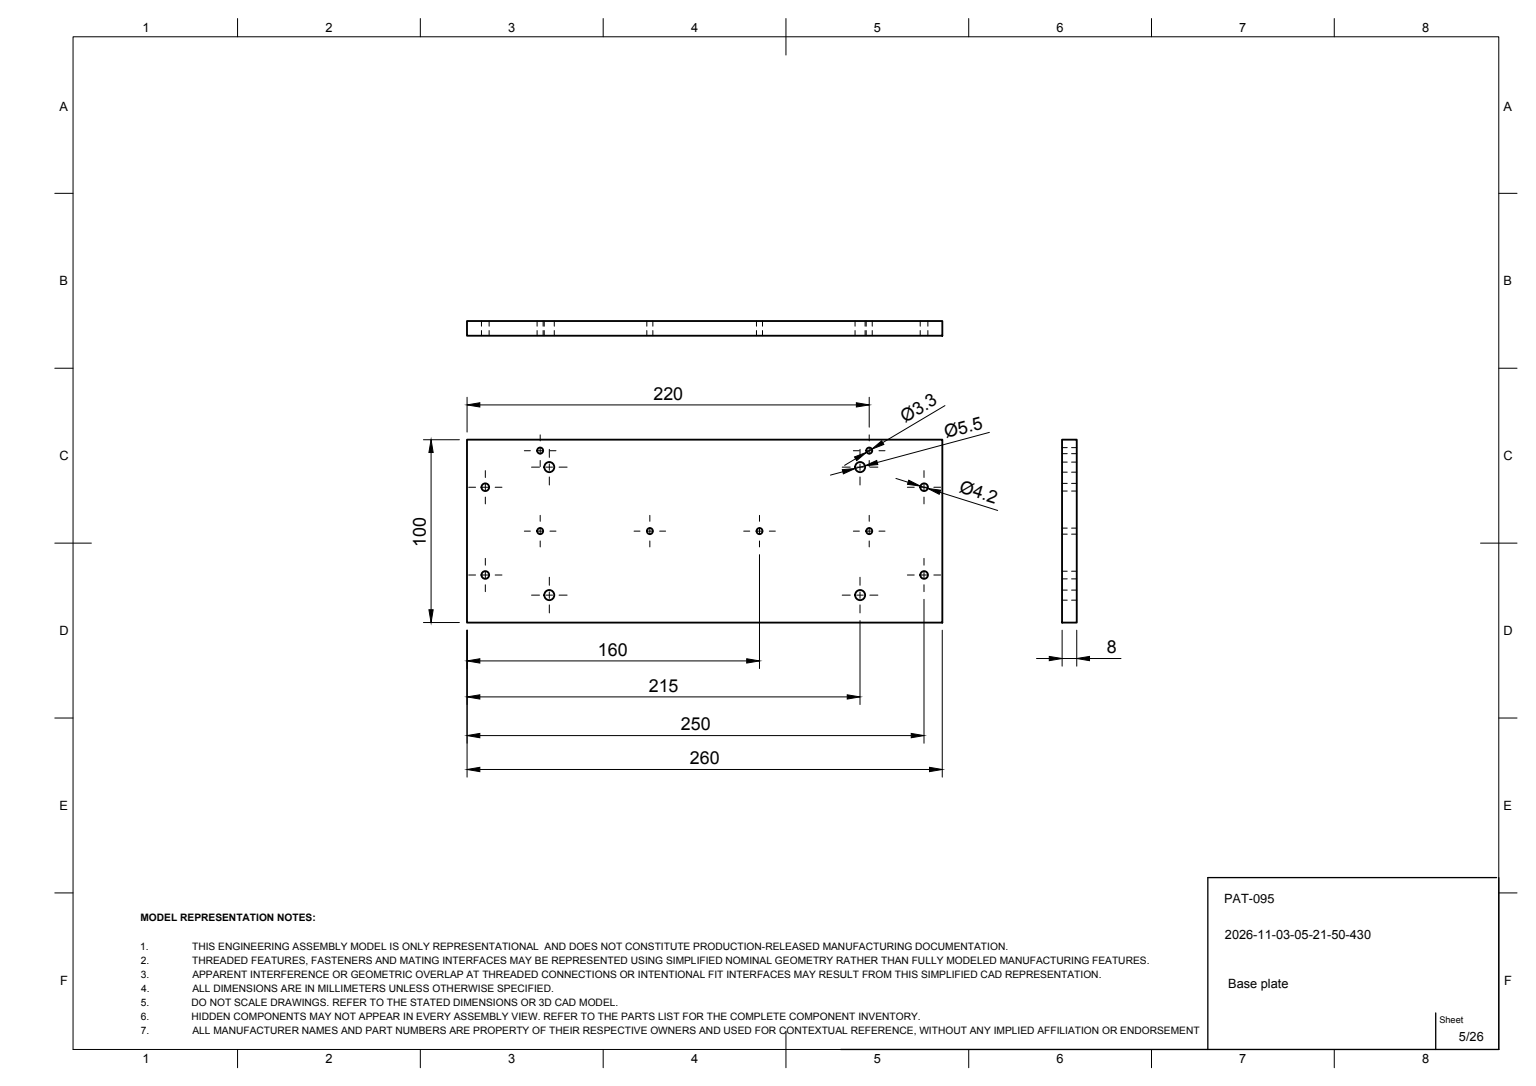
ISO-10303-21;
HEADER;
/* Generated by software containing ST-Developer
 * from STEP Tools, Inc. (www.steptools.com) 
 */

FILE_DESCRIPTION(
/* description */ ('Single-Axis Profile-Rail Linear Slide'),
/* implementation_level */ '2;1');

FILE_NAME(
/* name */ 'Base plate.step',
/* time_stamp */ '2026-10-27T10:47:43-07:00',
/* author */ (''),
/* organization */ (''),
/* preprocessor_version */ 'ST-DEVELOPER v20.2',
/* originating_system */ 'Autodesk Translation Framework v15.17.0.0',
/* authorisation */ '');

FILE_SCHEMA (('AUTOMOTIVE_DESIGN { 1 0 10303 214 3 1 1 }'));
ENDSEC;

DATA;
#10=MECHANICAL_DESIGN_GEOMETRIC_PRESENTATION_REPRESENTATION('',(#329),#14478);
#275=SHAPE_REPRESENTATION_RELATIONSHIP('SRR','None',#14605,#302);
#302=ADVANCED_BREP_SHAPE_REPRESENTATION('',(#356),#14449);
#329=STYLED_ITEM('',(#14810),#356);
#356=MANIFOLD_SOLID_BREP('Body1',#8589);
#378=FACE_BOUND('',#1314,.T.);
#379=FACE_BOUND('',#1315,.T.);
#380=FACE_BOUND('',#1316,.T.);
#381=FACE_BOUND('',#1317,.T.);
#382=FACE_BOUND('',#1318,.T.);
#383=FACE_BOUND('',#1319,.T.);
#384=FACE_BOUND('',#1320,.T.);
#385=FACE_BOUND('',#1321,.T.);
#386=FACE_BOUND('',#1322,.T.);
#387=FACE_BOUND('',#1323,.T.);
#388=FACE_BOUND('',#1324,.T.);
#389=FACE_BOUND('',#1325,.T.);
#390=FACE_BOUND('',#1326,.T.);
#391=FACE_BOUND('',#1327,.T.);
#392=FACE_BOUND('',#1329,.T.);
#393=FACE_BOUND('',#1330,.T.);
#394=FACE_BOUND('',#1331,.T.);
#395=FACE_BOUND('',#1332,.T.);
#396=FACE_BOUND('',#1333,.T.);
#397=FACE_BOUND('',#1334,.T.);
#398=FACE_BOUND('',#1335,.T.);
#399=FACE_BOUND('',#1336,.T.);
#400=FACE_BOUND('',#1337,.T.);
#401=FACE_BOUND('',#1338,.T.);
#402=FACE_BOUND('',#1339,.T.);
#403=FACE_BOUND('',#1340,.T.);
#404=FACE_BOUND('',#1341,.T.);
#405=FACE_BOUND('',#1342,.T.);
#468=PLANE('',#8964);
#469=PLANE('',#8965);
#470=PLANE('',#8966);
#471=PLANE('',#8967);
#472=PLANE('',#8968);
#473=PLANE('',#8969);
#840=FACE_OUTER_BOUND('',#1295,.T.);
#841=FACE_OUTER_BOUND('',#1296,.T.);
#842=FACE_OUTER_BOUND('',#1297,.T.);
#843=FACE_OUTER_BOUND('',#1298,.T.);
#844=FACE_OUTER_BOUND('',#1299,.T.);
#845=FACE_OUTER_BOUND('',#1300,.T.);
#846=FACE_OUTER_BOUND('',#1301,.T.);
#847=FACE_OUTER_BOUND('',#1302,.T.);
#848=FACE_OUTER_BOUND('',#1303,.T.);
#849=FACE_OUTER_BOUND('',#1304,.T.);
#850=FACE_OUTER_BOUND('',#1305,.T.);
#851=FACE_OUTER_BOUND('',#1306,.T.);
#852=FACE_OUTER_BOUND('',#1307,.T.);
#853=FACE_OUTER_BOUND('',#1308,.T.);
#854=FACE_OUTER_BOUND('',#1309,.T.);
#855=FACE_OUTER_BOUND('',#1310,.T.);
#856=FACE_OUTER_BOUND('',#1311,.T.);
#857=FACE_OUTER_BOUND('',#1312,.T.);
#858=FACE_OUTER_BOUND('',#1313,.T.);
#859=FACE_OUTER_BOUND('',#1328,.T.);
#1295=EDGE_LOOP('',(#5813,#5814,#5815,#5816));
#1296=EDGE_LOOP('',(#5817,#5818,#5819,#5820));
#1297=EDGE_LOOP('',(#5821,#5822,#5823,#5824));
#1298=EDGE_LOOP('',(#5825,#5826,#5827,#5828));
#1299=EDGE_LOOP('',(#5829,#5830,#5831,#5832));
#1300=EDGE_LOOP('',(#5833,#5834,#5835,#5836));
#1301=EDGE_LOOP('',(#5837,#5838,#5839,#5840));
#1302=EDGE_LOOP('',(#5841,#5842,#5843,#5844));
#1303=EDGE_LOOP('',(#5845,#5846,#5847,#5848));
#1304=EDGE_LOOP('',(#5849,#5850,#5851,#5852));
#1305=EDGE_LOOP('',(#5853,#5854,#5855,#5856));
#1306=EDGE_LOOP('',(#5857,#5858,#5859,#5860));
#1307=EDGE_LOOP('',(#5861,#5862,#5863,#5864));
#1308=EDGE_LOOP('',(#5865,#5866,#5867,#5868));
#1309=EDGE_LOOP('',(#5869,#5870,#5871,#5872));
#1310=EDGE_LOOP('',(#5873,#5874,#5875,#5876));
#1311=EDGE_LOOP('',(#5877,#5878,#5879,#5880));
#1312=EDGE_LOOP('',(#5881,#5882,#5883,#5884));
#1313=EDGE_LOOP('',(#5885,#5886,#5887,#5888));
#1314=EDGE_LOOP('',(#5889));
#1315=EDGE_LOOP('',(#5890));
#1316=EDGE_LOOP('',(#5891));
#1317=EDGE_LOOP('',(#5892));
#1318=EDGE_LOOP('',(#5893));
#1319=EDGE_LOOP('',(#5894));
#1320=EDGE_LOOP('',(#5895));
#1321=EDGE_LOOP('',(#5896));
#1322=EDGE_LOOP('',(#5897));
#1323=EDGE_LOOP('',(#5898));
#1324=EDGE_LOOP('',(#5899));
#1325=EDGE_LOOP('',(#5900));
#1326=EDGE_LOOP('',(#5901));
#1327=EDGE_LOOP('',(#5902));
#1328=EDGE_LOOP('',(#5903,#5904,#5905,#5906));
#1329=EDGE_LOOP('',(#5907));
#1330=EDGE_LOOP('',(#5908));
#1331=EDGE_LOOP('',(#5909));
#1332=EDGE_LOOP('',(#5910));
#1333=EDGE_LOOP('',(#5911));
#1334=EDGE_LOOP('',(#5912));
#1335=EDGE_LOOP('',(#5913));
#1336=EDGE_LOOP('',(#5914));
#1337=EDGE_LOOP('',(#5915));
#1338=EDGE_LOOP('',(#5916));
#1339=EDGE_LOOP('',(#5917));
#1340=EDGE_LOOP('',(#5918));
#1341=EDGE_LOOP('',(#5919));
#1342=EDGE_LOOP('',(#5920));
#1840=LINE('',#12003,#2811);
#1841=LINE('',#12009,#2812);
#1842=LINE('',#12015,#2813);
#1843=LINE('',#12021,#2814);
#1844=LINE('',#12027,#2815);
#1845=LINE('',#12033,#2816);
#1846=LINE('',#12039,#2817);
#1847=LINE('',#12045,#2818);
#1848=LINE('',#12051,#2819);
#1849=LINE('',#12057,#2820);
#1850=LINE('',#12063,#2821);
#1851=LINE('',#12069,#2822);
#1852=LINE('',#12075,#2823);
#1853=LINE('',#12081,#2824);
#1854=LINE('',#12086,#2825);
#1855=LINE('',#12088,#2826);
#1856=LINE('',#12090,#2827);
#1857=LINE('',#12091,#2828);
#1858=LINE('',#12094,#2829);
#1859=LINE('',#12096,#2830);
#1860=LINE('',#12097,#2831);
#1861=LINE('',#12100,#2832);
#1862=LINE('',#12102,#2833);
#1863=LINE('',#12103,#2834);
#1864=LINE('',#12105,#2835);
#1865=LINE('',#12106,#2836);
#2811=VECTOR('',#9631,0.165);
#2812=VECTOR('',#9638,0.164999999999999);
#2813=VECTOR('',#9645,0.210000000000001);
#2814=VECTOR('',#9652,0.21);
#2815=VECTOR('',#9659,0.21);
#2816=VECTOR('',#9666,0.210000000000001);
#2817=VECTOR('',#9673,0.274999999999999);
#2818=VECTOR('',#9680,0.275);
#2819=VECTOR('',#9687,0.275);
#2820=VECTOR('',#9694,0.274999999999999);
#2821=VECTOR('',#9701,0.164999999999999);
#2822=VECTOR('',#9708,0.164999999999999);
#2823=VECTOR('',#9715,0.165);
#2824=VECTOR('',#9722,0.164999999999999);
#2825=VECTOR('',#9727,1.);
#2826=VECTOR('',#9728,1.);
#2827=VECTOR('',#9729,1.);
#2828=VECTOR('',#9730,1.);
#2829=VECTOR('',#9733,1.);
#2830=VECTOR('',#9734,1.);
#2831=VECTOR('',#9735,1.);
#2832=VECTOR('',#9738,1.);
#2833=VECTOR('',#9739,1.);
#2834=VECTOR('',#9740,1.);
#2835=VECTOR('',#9743,1.);
#2836=VECTOR('',#9744,1.);
#3782=CIRCLE('',#8923,0.165);
#3783=CIRCLE('',#8924,0.165);
#3784=CIRCLE('',#8926,0.164999999999999);
#3785=CIRCLE('',#8927,0.164999999999999);
#3786=CIRCLE('',#8929,0.210000000000001);
#3787=CIRCLE('',#8930,0.210000000000001);
#3788=CIRCLE('',#8932,0.21);
#3789=CIRCLE('',#8933,0.21);
#3790=CIRCLE('',#8935,0.21);
#3791=CIRCLE('',#8936,0.21);
#3792=CIRCLE('',#8938,0.210000000000001);
#3793=CIRCLE('',#8939,0.210000000000001);
#3794=CIRCLE('',#8941,0.274999999999999);
#3795=CIRCLE('',#8942,0.274999999999999);
#3796=CIRCLE('',#8944,0.275);
#3797=CIRCLE('',#8945,0.275);
#3798=CIRCLE('',#8947,0.275);
#3799=CIRCLE('',#8948,0.275);
#3800=CIRCLE('',#8950,0.274999999999999);
#3801=CIRCLE('',#8951,0.274999999999999);
#3802=CIRCLE('',#8953,0.164999999999999);
#3803=CIRCLE('',#8954,0.164999999999999);
#3804=CIRCLE('',#8956,0.164999999999999);
#3805=CIRCLE('',#8957,0.164999999999999);
#3806=CIRCLE('',#8959,0.165);
#3807=CIRCLE('',#8960,0.165);
#3808=CIRCLE('',#8962,0.164999999999999);
#3809=CIRCLE('',#8963,0.164999999999999);
#3938=VERTEX_POINT('',#12000);
#3939=VERTEX_POINT('',#12002);
#3940=VERTEX_POINT('',#12006);
#3941=VERTEX_POINT('',#12008);
#3942=VERTEX_POINT('',#12012);
#3943=VERTEX_POINT('',#12014);
#3944=VERTEX_POINT('',#12018);
#3945=VERTEX_POINT('',#12020);
#3946=VERTEX_POINT('',#12024);
#3947=VERTEX_POINT('',#12026);
#3948=VERTEX_POINT('',#12030);
#3949=VERTEX_POINT('',#12032);
#3950=VERTEX_POINT('',#12036);
#3951=VERTEX_POINT('',#12038);
#3952=VERTEX_POINT('',#12042);
#3953=VERTEX_POINT('',#12044);
#3954=VERTEX_POINT('',#12048);
#3955=VERTEX_POINT('',#12050);
#3956=VERTEX_POINT('',#12054);
#3957=VERTEX_POINT('',#12056);
#3958=VERTEX_POINT('',#12060);
#3959=VERTEX_POINT('',#12062);
#3960=VERTEX_POINT('',#12066);
#3961=VERTEX_POINT('',#12068);
#3962=VERTEX_POINT('',#12072);
#3963=VERTEX_POINT('',#12074);
#3964=VERTEX_POINT('',#12078);
#3965=VERTEX_POINT('',#12080);
#3966=VERTEX_POINT('',#12084);
#3967=VERTEX_POINT('',#12085);
#3968=VERTEX_POINT('',#12087);
#3969=VERTEX_POINT('',#12089);
#3970=VERTEX_POINT('',#12093);
#3971=VERTEX_POINT('',#12095);
#3972=VERTEX_POINT('',#12099);
#3973=VERTEX_POINT('',#12101);
#4684=EDGE_CURVE('',#3938,#3938,#3782,.T.);
#4685=EDGE_CURVE('',#3938,#3939,#1840,.T.);
#4686=EDGE_CURVE('',#3939,#3939,#3783,.T.);
#4687=EDGE_CURVE('',#3940,#3940,#3784,.T.);
#4688=EDGE_CURVE('',#3940,#3941,#1841,.T.);
#4689=EDGE_CURVE('',#3941,#3941,#3785,.T.);
#4690=EDGE_CURVE('',#3942,#3942,#3786,.T.);
#4691=EDGE_CURVE('',#3942,#3943,#1842,.T.);
#4692=EDGE_CURVE('',#3943,#3943,#3787,.T.);
#4693=EDGE_CURVE('',#3944,#3944,#3788,.T.);
#4694=EDGE_CURVE('',#3944,#3945,#1843,.T.);
#4695=EDGE_CURVE('',#3945,#3945,#3789,.T.);
#4696=EDGE_CURVE('',#3946,#3946,#3790,.T.);
#4697=EDGE_CURVE('',#3946,#3947,#1844,.T.);
#4698=EDGE_CURVE('',#3947,#3947,#3791,.T.);
#4699=EDGE_CURVE('',#3948,#3948,#3792,.T.);
#4700=EDGE_CURVE('',#3948,#3949,#1845,.T.);
#4701=EDGE_CURVE('',#3949,#3949,#3793,.T.);
#4702=EDGE_CURVE('',#3950,#3950,#3794,.T.);
#4703=EDGE_CURVE('',#3950,#3951,#1846,.T.);
#4704=EDGE_CURVE('',#3951,#3951,#3795,.T.);
#4705=EDGE_CURVE('',#3952,#3952,#3796,.T.);
#4706=EDGE_CURVE('',#3952,#3953,#1847,.T.);
#4707=EDGE_CURVE('',#3953,#3953,#3797,.T.);
#4708=EDGE_CURVE('',#3954,#3954,#3798,.T.);
#4709=EDGE_CURVE('',#3954,#3955,#1848,.T.);
#4710=EDGE_CURVE('',#3955,#3955,#3799,.T.);
#4711=EDGE_CURVE('',#3956,#3956,#3800,.T.);
#4712=EDGE_CURVE('',#3956,#3957,#1849,.T.);
#4713=EDGE_CURVE('',#3957,#3957,#3801,.T.);
#4714=EDGE_CURVE('',#3958,#3958,#3802,.T.);
#4715=EDGE_CURVE('',#3958,#3959,#1850,.T.);
#4716=EDGE_CURVE('',#3959,#3959,#3803,.T.);
#4717=EDGE_CURVE('',#3960,#3960,#3804,.T.);
#4718=EDGE_CURVE('',#3960,#3961,#1851,.T.);
#4719=EDGE_CURVE('',#3961,#3961,#3805,.T.);
#4720=EDGE_CURVE('',#3962,#3962,#3806,.T.);
#4721=EDGE_CURVE('',#3962,#3963,#1852,.T.);
#4722=EDGE_CURVE('',#3963,#3963,#3807,.T.);
#4723=EDGE_CURVE('',#3964,#3964,#3808,.T.);
#4724=EDGE_CURVE('',#3964,#3965,#1853,.T.);
#4725=EDGE_CURVE('',#3965,#3965,#3809,.T.);
#4726=EDGE_CURVE('',#3966,#3967,#1854,.T.);
#4727=EDGE_CURVE('',#3967,#3968,#1855,.T.);
#4728=EDGE_CURVE('',#3969,#3968,#1856,.T.);
#4729=EDGE_CURVE('',#3966,#3969,#1857,.T.);
#4730=EDGE_CURVE('',#3970,#3966,#1858,.T.);
#4731=EDGE_CURVE('',#3971,#3969,#1859,.T.);
#4732=EDGE_CURVE('',#3970,#3971,#1860,.T.);
#4733=EDGE_CURVE('',#3972,#3970,#1861,.T.);
#4734=EDGE_CURVE('',#3973,#3971,#1862,.T.);
#4735=EDGE_CURVE('',#3972,#3973,#1863,.T.);
#4736=EDGE_CURVE('',#3967,#3972,#1864,.T.);
#4737=EDGE_CURVE('',#3968,#3973,#1865,.T.);
#5813=ORIENTED_EDGE('',*,*,#4684,.F.);
#5814=ORIENTED_EDGE('',*,*,#4685,.T.);
#5815=ORIENTED_EDGE('',*,*,#4686,.F.);
#5816=ORIENTED_EDGE('',*,*,#4685,.F.);
#5817=ORIENTED_EDGE('',*,*,#4687,.F.);
#5818=ORIENTED_EDGE('',*,*,#4688,.T.);
#5819=ORIENTED_EDGE('',*,*,#4689,.F.);
#5820=ORIENTED_EDGE('',*,*,#4688,.F.);
#5821=ORIENTED_EDGE('',*,*,#4690,.F.);
#5822=ORIENTED_EDGE('',*,*,#4691,.T.);
#5823=ORIENTED_EDGE('',*,*,#4692,.F.);
#5824=ORIENTED_EDGE('',*,*,#4691,.F.);
#5825=ORIENTED_EDGE('',*,*,#4693,.F.);
#5826=ORIENTED_EDGE('',*,*,#4694,.T.);
#5827=ORIENTED_EDGE('',*,*,#4695,.F.);
#5828=ORIENTED_EDGE('',*,*,#4694,.F.);
#5829=ORIENTED_EDGE('',*,*,#4696,.F.);
#5830=ORIENTED_EDGE('',*,*,#4697,.T.);
#5831=ORIENTED_EDGE('',*,*,#4698,.F.);
#5832=ORIENTED_EDGE('',*,*,#4697,.F.);
#5833=ORIENTED_EDGE('',*,*,#4699,.F.);
#5834=ORIENTED_EDGE('',*,*,#4700,.T.);
#5835=ORIENTED_EDGE('',*,*,#4701,.F.);
#5836=ORIENTED_EDGE('',*,*,#4700,.F.);
#5837=ORIENTED_EDGE('',*,*,#4702,.F.);
#5838=ORIENTED_EDGE('',*,*,#4703,.T.);
#5839=ORIENTED_EDGE('',*,*,#4704,.F.);
#5840=ORIENTED_EDGE('',*,*,#4703,.F.);
#5841=ORIENTED_EDGE('',*,*,#4705,.F.);
#5842=ORIENTED_EDGE('',*,*,#4706,.T.);
#5843=ORIENTED_EDGE('',*,*,#4707,.F.);
#5844=ORIENTED_EDGE('',*,*,#4706,.F.);
#5845=ORIENTED_EDGE('',*,*,#4708,.F.);
#5846=ORIENTED_EDGE('',*,*,#4709,.T.);
#5847=ORIENTED_EDGE('',*,*,#4710,.F.);
#5848=ORIENTED_EDGE('',*,*,#4709,.F.);
#5849=ORIENTED_EDGE('',*,*,#4711,.F.);
#5850=ORIENTED_EDGE('',*,*,#4712,.T.);
#5851=ORIENTED_EDGE('',*,*,#4713,.F.);
#5852=ORIENTED_EDGE('',*,*,#4712,.F.);
#5853=ORIENTED_EDGE('',*,*,#4714,.F.);
#5854=ORIENTED_EDGE('',*,*,#4715,.T.);
#5855=ORIENTED_EDGE('',*,*,#4716,.F.);
#5856=ORIENTED_EDGE('',*,*,#4715,.F.);
#5857=ORIENTED_EDGE('',*,*,#4717,.F.);
#5858=ORIENTED_EDGE('',*,*,#4718,.T.);
#5859=ORIENTED_EDGE('',*,*,#4719,.F.);
#5860=ORIENTED_EDGE('',*,*,#4718,.F.);
#5861=ORIENTED_EDGE('',*,*,#4720,.F.);
#5862=ORIENTED_EDGE('',*,*,#4721,.T.);
#5863=ORIENTED_EDGE('',*,*,#4722,.F.);
#5864=ORIENTED_EDGE('',*,*,#4721,.F.);
#5865=ORIENTED_EDGE('',*,*,#4723,.F.);
#5866=ORIENTED_EDGE('',*,*,#4724,.T.);
#5867=ORIENTED_EDGE('',*,*,#4725,.F.);
#5868=ORIENTED_EDGE('',*,*,#4724,.F.);
#5869=ORIENTED_EDGE('',*,*,#4726,.T.);
#5870=ORIENTED_EDGE('',*,*,#4727,.T.);
#5871=ORIENTED_EDGE('',*,*,#4728,.F.);
#5872=ORIENTED_EDGE('',*,*,#4729,.F.);
#5873=ORIENTED_EDGE('',*,*,#4730,.T.);
#5874=ORIENTED_EDGE('',*,*,#4729,.T.);
#5875=ORIENTED_EDGE('',*,*,#4731,.F.);
#5876=ORIENTED_EDGE('',*,*,#4732,.F.);
#5877=ORIENTED_EDGE('',*,*,#4733,.T.);
#5878=ORIENTED_EDGE('',*,*,#4732,.T.);
#5879=ORIENTED_EDGE('',*,*,#4734,.F.);
#5880=ORIENTED_EDGE('',*,*,#4735,.F.);
#5881=ORIENTED_EDGE('',*,*,#4736,.T.);
#5882=ORIENTED_EDGE('',*,*,#4735,.T.);
#5883=ORIENTED_EDGE('',*,*,#4737,.F.);
#5884=ORIENTED_EDGE('',*,*,#4727,.F.);
#5885=ORIENTED_EDGE('',*,*,#4737,.T.);
#5886=ORIENTED_EDGE('',*,*,#4734,.T.);
#5887=ORIENTED_EDGE('',*,*,#4731,.T.);
#5888=ORIENTED_EDGE('',*,*,#4728,.T.);
#5889=ORIENTED_EDGE('',*,*,#4692,.T.);
#5890=ORIENTED_EDGE('',*,*,#4695,.T.);
#5891=ORIENTED_EDGE('',*,*,#4698,.T.);
#5892=ORIENTED_EDGE('',*,*,#4701,.T.);
#5893=ORIENTED_EDGE('',*,*,#4725,.T.);
#5894=ORIENTED_EDGE('',*,*,#4722,.T.);
#5895=ORIENTED_EDGE('',*,*,#4719,.T.);
#5896=ORIENTED_EDGE('',*,*,#4716,.T.);
#5897=ORIENTED_EDGE('',*,*,#4713,.T.);
#5898=ORIENTED_EDGE('',*,*,#4710,.T.);
#5899=ORIENTED_EDGE('',*,*,#4707,.T.);
#5900=ORIENTED_EDGE('',*,*,#4704,.T.);
#5901=ORIENTED_EDGE('',*,*,#4689,.T.);
#5902=ORIENTED_EDGE('',*,*,#4686,.T.);
#5903=ORIENTED_EDGE('',*,*,#4736,.F.);
#5904=ORIENTED_EDGE('',*,*,#4726,.F.);
#5905=ORIENTED_EDGE('',*,*,#4730,.F.);
#5906=ORIENTED_EDGE('',*,*,#4733,.F.);
#5907=ORIENTED_EDGE('',*,*,#4690,.T.);
#5908=ORIENTED_EDGE('',*,*,#4693,.T.);
#5909=ORIENTED_EDGE('',*,*,#4696,.T.);
#5910=ORIENTED_EDGE('',*,*,#4699,.T.);
#5911=ORIENTED_EDGE('',*,*,#4723,.T.);
#5912=ORIENTED_EDGE('',*,*,#4720,.T.);
#5913=ORIENTED_EDGE('',*,*,#4717,.T.);
#5914=ORIENTED_EDGE('',*,*,#4714,.T.);
#5915=ORIENTED_EDGE('',*,*,#4711,.T.);
#5916=ORIENTED_EDGE('',*,*,#4708,.T.);
#5917=ORIENTED_EDGE('',*,*,#4705,.T.);
#5918=ORIENTED_EDGE('',*,*,#4702,.T.);
#5919=ORIENTED_EDGE('',*,*,#4687,.T.);
#5920=ORIENTED_EDGE('',*,*,#4684,.T.);
#8071=CYLINDRICAL_SURFACE('',#8922,0.165);
#8072=CYLINDRICAL_SURFACE('',#8925,0.164999999999999);
#8073=CYLINDRICAL_SURFACE('',#8928,0.210000000000001);
#8074=CYLINDRICAL_SURFACE('',#8931,0.21);
#8075=CYLINDRICAL_SURFACE('',#8934,0.21);
#8076=CYLINDRICAL_SURFACE('',#8937,0.210000000000001);
#8077=CYLINDRICAL_SURFACE('',#8940,0.274999999999999);
#8078=CYLINDRICAL_SURFACE('',#8943,0.275);
#8079=CYLINDRICAL_SURFACE('',#8946,0.275);
#8080=CYLINDRICAL_SURFACE('',#8949,0.274999999999999);
#8081=CYLINDRICAL_SURFACE('',#8952,0.164999999999999);
#8082=CYLINDRICAL_SURFACE('',#8955,0.164999999999999);
#8083=CYLINDRICAL_SURFACE('',#8958,0.165);
#8084=CYLINDRICAL_SURFACE('',#8961,0.164999999999999);
#8134=ADVANCED_FACE('',(#840),#8071,.F.);
#8135=ADVANCED_FACE('',(#841),#8072,.F.);
#8136=ADVANCED_FACE('',(#842),#8073,.F.);
#8137=ADVANCED_FACE('',(#843),#8074,.F.);
#8138=ADVANCED_FACE('',(#844),#8075,.F.);
#8139=ADVANCED_FACE('',(#845),#8076,.F.);
#8140=ADVANCED_FACE('',(#846),#8077,.F.);
#8141=ADVANCED_FACE('',(#847),#8078,.F.);
#8142=ADVANCED_FACE('',(#848),#8079,.F.);
#8143=ADVANCED_FACE('',(#849),#8080,.F.);
#8144=ADVANCED_FACE('',(#850),#8081,.F.);
#8145=ADVANCED_FACE('',(#851),#8082,.F.);
#8146=ADVANCED_FACE('',(#852),#8083,.F.);
#8147=ADVANCED_FACE('',(#853),#8084,.F.);
#8148=ADVANCED_FACE('',(#854),#468,.T.);
#8149=ADVANCED_FACE('',(#855),#469,.T.);
#8150=ADVANCED_FACE('',(#856),#470,.T.);
#8151=ADVANCED_FACE('',(#857),#471,.T.);
#8152=ADVANCED_FACE('',(#858,#378,#379,#380,#381,#382,#383,#384,#385,#386,
#387,#388,#389,#390,#391),#472,.T.);
#8153=ADVANCED_FACE('',(#859,#392,#393,#394,#395,#396,#397,#398,#399,#400,
#401,#402,#403,#404,#405),#473,.F.);
#8589=CLOSED_SHELL('',(#8134,#8135,#8136,#8137,#8138,#8139,#8140,#8141,
#8142,#8143,#8144,#8145,#8146,#8147,#8148,#8149,#8150,#8151,#8152,#8153));
#8921=AXIS2_PLACEMENT_3D('',#11998,#9625,#9626);
#8922=AXIS2_PLACEMENT_3D('',#11999,#9627,#9628);
#8923=AXIS2_PLACEMENT_3D('',#12001,#9629,#9630);
#8924=AXIS2_PLACEMENT_3D('',#12004,#9632,#9633);
#8925=AXIS2_PLACEMENT_3D('',#12005,#9634,#9635);
#8926=AXIS2_PLACEMENT_3D('',#12007,#9636,#9637);
#8927=AXIS2_PLACEMENT_3D('',#12010,#9639,#9640);
#8928=AXIS2_PLACEMENT_3D('',#12011,#9641,#9642);
#8929=AXIS2_PLACEMENT_3D('',#12013,#9643,#9644);
#8930=AXIS2_PLACEMENT_3D('',#12016,#9646,#9647);
#8931=AXIS2_PLACEMENT_3D('',#12017,#9648,#9649);
#8932=AXIS2_PLACEMENT_3D('',#12019,#9650,#9651);
#8933=AXIS2_PLACEMENT_3D('',#12022,#9653,#9654);
#8934=AXIS2_PLACEMENT_3D('',#12023,#9655,#9656);
#8935=AXIS2_PLACEMENT_3D('',#12025,#9657,#9658);
#8936=AXIS2_PLACEMENT_3D('',#12028,#9660,#9661);
#8937=AXIS2_PLACEMENT_3D('',#12029,#9662,#9663);
#8938=AXIS2_PLACEMENT_3D('',#12031,#9664,#9665);
#8939=AXIS2_PLACEMENT_3D('',#12034,#9667,#9668);
#8940=AXIS2_PLACEMENT_3D('',#12035,#9669,#9670);
#8941=AXIS2_PLACEMENT_3D('',#12037,#9671,#9672);
#8942=AXIS2_PLACEMENT_3D('',#12040,#9674,#9675);
#8943=AXIS2_PLACEMENT_3D('',#12041,#9676,#9677);
#8944=AXIS2_PLACEMENT_3D('',#12043,#9678,#9679);
#8945=AXIS2_PLACEMENT_3D('',#12046,#9681,#9682);
#8946=AXIS2_PLACEMENT_3D('',#12047,#9683,#9684);
#8947=AXIS2_PLACEMENT_3D('',#12049,#9685,#9686);
#8948=AXIS2_PLACEMENT_3D('',#12052,#9688,#9689);
#8949=AXIS2_PLACEMENT_3D('',#12053,#9690,#9691);
#8950=AXIS2_PLACEMENT_3D('',#12055,#9692,#9693);
#8951=AXIS2_PLACEMENT_3D('',#12058,#9695,#9696);
#8952=AXIS2_PLACEMENT_3D('',#12059,#9697,#9698);
#8953=AXIS2_PLACEMENT_3D('',#12061,#9699,#9700);
#8954=AXIS2_PLACEMENT_3D('',#12064,#9702,#9703);
#8955=AXIS2_PLACEMENT_3D('',#12065,#9704,#9705);
#8956=AXIS2_PLACEMENT_3D('',#12067,#9706,#9707);
#8957=AXIS2_PLACEMENT_3D('',#12070,#9709,#9710);
#8958=AXIS2_PLACEMENT_3D('',#12071,#9711,#9712);
#8959=AXIS2_PLACEMENT_3D('',#12073,#9713,#9714);
#8960=AXIS2_PLACEMENT_3D('',#12076,#9716,#9717);
#8961=AXIS2_PLACEMENT_3D('',#12077,#9718,#9719);
#8962=AXIS2_PLACEMENT_3D('',#12079,#9720,#9721);
#8963=AXIS2_PLACEMENT_3D('',#12082,#9723,#9724);
#8964=AXIS2_PLACEMENT_3D('',#12083,#9725,#9726);
#8965=AXIS2_PLACEMENT_3D('',#12092,#9731,#9732);
#8966=AXIS2_PLACEMENT_3D('',#12098,#9736,#9737);
#8967=AXIS2_PLACEMENT_3D('',#12104,#9741,#9742);
#8968=AXIS2_PLACEMENT_3D('',#12107,#9745,#9746);
#8969=AXIS2_PLACEMENT_3D('',#12108,#9747,#9748);
#9625=DIRECTION('axis',(0.,0.,1.));
#9626=DIRECTION('refdir',(1.,0.,0.));
#9627=DIRECTION('center_axis',(0.,0.,1.));
#9628=DIRECTION('ref_axis',(1.,0.,0.));
#9629=DIRECTION('center_axis',(0.,0.,1.));
#9630=DIRECTION('ref_axis',(1.,0.,0.));
#9631=DIRECTION('',(0.,0.,1.));
#9632=DIRECTION('center_axis',(0.,0.,-1.));
#9633=DIRECTION('ref_axis',(1.,0.,0.));
#9634=DIRECTION('center_axis',(0.,0.,1.));
#9635=DIRECTION('ref_axis',(1.,0.,0.));
#9636=DIRECTION('center_axis',(0.,0.,1.));
#9637=DIRECTION('ref_axis',(1.,0.,0.));
#9638=DIRECTION('',(0.,0.,1.));
#9639=DIRECTION('center_axis',(0.,0.,-1.));
#9640=DIRECTION('ref_axis',(1.,0.,0.));
#9641=DIRECTION('center_axis',(0.,0.,1.));
#9642=DIRECTION('ref_axis',(1.,0.,0.));
#9643=DIRECTION('center_axis',(0.,0.,1.));
#9644=DIRECTION('ref_axis',(1.,0.,0.));
#9645=DIRECTION('',(0.,0.,1.));
#9646=DIRECTION('center_axis',(0.,0.,-1.));
#9647=DIRECTION('ref_axis',(1.,0.,0.));
#9648=DIRECTION('center_axis',(0.,0.,1.));
#9649=DIRECTION('ref_axis',(1.,0.,0.));
#9650=DIRECTION('center_axis',(0.,0.,1.));
#9651=DIRECTION('ref_axis',(1.,0.,0.));
#9652=DIRECTION('',(0.,0.,1.));
#9653=DIRECTION('center_axis',(0.,0.,-1.));
#9654=DIRECTION('ref_axis',(1.,0.,0.));
#9655=DIRECTION('center_axis',(0.,0.,1.));
#9656=DIRECTION('ref_axis',(1.,0.,0.));
#9657=DIRECTION('center_axis',(0.,0.,1.));
#9658=DIRECTION('ref_axis',(1.,0.,0.));
#9659=DIRECTION('',(0.,0.,1.));
#9660=DIRECTION('center_axis',(0.,0.,-1.));
#9661=DIRECTION('ref_axis',(1.,0.,0.));
#9662=DIRECTION('center_axis',(0.,0.,1.));
#9663=DIRECTION('ref_axis',(1.,0.,0.));
#9664=DIRECTION('center_axis',(0.,0.,1.));
#9665=DIRECTION('ref_axis',(1.,0.,0.));
#9666=DIRECTION('',(0.,0.,1.));
#9667=DIRECTION('center_axis',(0.,0.,-1.));
#9668=DIRECTION('ref_axis',(1.,0.,0.));
#9669=DIRECTION('center_axis',(0.,0.,1.));
#9670=DIRECTION('ref_axis',(1.,0.,0.));
#9671=DIRECTION('center_axis',(0.,0.,1.));
#9672=DIRECTION('ref_axis',(1.,0.,0.));
#9673=DIRECTION('',(0.,0.,1.));
#9674=DIRECTION('center_axis',(0.,0.,-1.));
#9675=DIRECTION('ref_axis',(1.,0.,0.));
#9676=DIRECTION('center_axis',(0.,0.,1.));
#9677=DIRECTION('ref_axis',(1.,0.,0.));
#9678=DIRECTION('center_axis',(0.,0.,1.));
#9679=DIRECTION('ref_axis',(1.,0.,0.));
#9680=DIRECTION('',(0.,0.,1.));
#9681=DIRECTION('center_axis',(0.,0.,-1.));
#9682=DIRECTION('ref_axis',(1.,0.,0.));
#9683=DIRECTION('center_axis',(0.,0.,1.));
#9684=DIRECTION('ref_axis',(1.,0.,0.));
#9685=DIRECTION('center_axis',(0.,0.,1.));
#9686=DIRECTION('ref_axis',(1.,0.,0.));
#9687=DIRECTION('',(0.,0.,1.));
#9688=DIRECTION('center_axis',(0.,0.,-1.));
#9689=DIRECTION('ref_axis',(1.,0.,0.));
#9690=DIRECTION('center_axis',(0.,0.,1.));
#9691=DIRECTION('ref_axis',(1.,0.,0.));
#9692=DIRECTION('center_axis',(0.,0.,1.));
#9693=DIRECTION('ref_axis',(1.,0.,0.));
#9694=DIRECTION('',(0.,0.,1.));
#9695=DIRECTION('center_axis',(0.,0.,-1.));
#9696=DIRECTION('ref_axis',(1.,0.,0.));
#9697=DIRECTION('center_axis',(0.,0.,1.));
#9698=DIRECTION('ref_axis',(1.,0.,0.));
#9699=DIRECTION('center_axis',(0.,0.,1.));
#9700=DIRECTION('ref_axis',(1.,0.,0.));
#9701=DIRECTION('',(0.,0.,1.));
#9702=DIRECTION('center_axis',(0.,0.,-1.));
#9703=DIRECTION('ref_axis',(1.,0.,0.));
#9704=DIRECTION('center_axis',(0.,0.,1.));
#9705=DIRECTION('ref_axis',(1.,0.,0.));
#9706=DIRECTION('center_axis',(0.,0.,1.));
#9707=DIRECTION('ref_axis',(1.,0.,0.));
#9708=DIRECTION('',(0.,0.,1.));
#9709=DIRECTION('center_axis',(0.,0.,-1.));
#9710=DIRECTION('ref_axis',(1.,0.,0.));
#9711=DIRECTION('center_axis',(0.,0.,1.));
#9712=DIRECTION('ref_axis',(1.,0.,0.));
#9713=DIRECTION('center_axis',(0.,0.,1.));
#9714=DIRECTION('ref_axis',(1.,0.,0.));
#9715=DIRECTION('',(0.,0.,1.));
#9716=DIRECTION('center_axis',(0.,0.,-1.));
#9717=DIRECTION('ref_axis',(1.,0.,0.));
#9718=DIRECTION('center_axis',(0.,0.,1.));
#9719=DIRECTION('ref_axis',(1.,0.,0.));
#9720=DIRECTION('center_axis',(0.,0.,1.));
#9721=DIRECTION('ref_axis',(1.,0.,0.));
#9722=DIRECTION('',(0.,0.,1.));
#9723=DIRECTION('center_axis',(0.,0.,-1.));
#9724=DIRECTION('ref_axis',(1.,0.,0.));
#9725=DIRECTION('center_axis',(0.,1.,0.));
#9726=DIRECTION('ref_axis',(-1.,0.,0.));
#9727=DIRECTION('',(-1.,0.,0.));
#9728=DIRECTION('',(0.,0.,1.));
#9729=DIRECTION('',(-1.,0.,0.));
#9730=DIRECTION('',(0.,0.,1.));
#9731=DIRECTION('center_axis',(1.,0.,0.));
#9732=DIRECTION('ref_axis',(0.,1.,0.));
#9733=DIRECTION('',(0.,1.,0.));
#9734=DIRECTION('',(0.,1.,0.));
#9735=DIRECTION('',(0.,0.,1.));
#9736=DIRECTION('center_axis',(0.,-1.,0.));
#9737=DIRECTION('ref_axis',(1.,0.,0.));
#9738=DIRECTION('',(1.,0.,0.));
#9739=DIRECTION('',(1.,0.,0.));
#9740=DIRECTION('',(0.,0.,1.));
#9741=DIRECTION('center_axis',(-1.,0.,0.));
#9742=DIRECTION('ref_axis',(0.,-1.,0.));
#9743=DIRECTION('',(0.,-1.,0.));
#9744=DIRECTION('',(0.,-1.,0.));
#9745=DIRECTION('center_axis',(0.,0.,1.));
#9746=DIRECTION('ref_axis',(1.,0.,0.));
#9747=DIRECTION('center_axis',(0.,0.,1.));
#9748=DIRECTION('ref_axis',(1.,0.,0.));
#11998=CARTESIAN_POINT('',(0.,0.,0.));
#11999=CARTESIAN_POINT('Origin',(2.,4.4,1.9));
#12000=CARTESIAN_POINT('',(1.835,4.4,2.));
#12001=CARTESIAN_POINT('Origin',(2.,4.4,2.));
#12002=CARTESIAN_POINT('',(1.835,4.4,2.8));
#12003=CARTESIAN_POINT('',(1.835,4.4,1.9));
#12004=CARTESIAN_POINT('Origin',(2.,4.4,2.8));
#12005=CARTESIAN_POINT('Origin',(20.,4.4,1.9));
#12006=CARTESIAN_POINT('',(19.835,4.4,2.));
#12007=CARTESIAN_POINT('Origin',(20.,4.4,2.));
#12008=CARTESIAN_POINT('',(19.835,4.4,2.8));
#12009=CARTESIAN_POINT('',(19.835,4.4,1.9));
#12010=CARTESIAN_POINT('Origin',(20.,4.4,2.8));
#12011=CARTESIAN_POINT('Origin',(23.,-2.4,1.9));
#12012=CARTESIAN_POINT('',(22.79,-2.4,2.));
#12013=CARTESIAN_POINT('Origin',(23.,-2.4,2.));
#12014=CARTESIAN_POINT('',(22.79,-2.4,2.8));
#12015=CARTESIAN_POINT('',(22.79,-2.4,1.9));
#12016=CARTESIAN_POINT('Origin',(23.,-2.4,2.8));
#12017=CARTESIAN_POINT('Origin',(-1.,2.4,1.9));
#12018=CARTESIAN_POINT('',(-1.21,2.4,2.));
#12019=CARTESIAN_POINT('Origin',(-1.,2.4,2.));
#12020=CARTESIAN_POINT('',(-1.21,2.4,2.8));
#12021=CARTESIAN_POINT('',(-1.21,2.4,1.9));
#12022=CARTESIAN_POINT('Origin',(-1.,2.4,2.8));
#12023=CARTESIAN_POINT('Origin',(-1.,-2.4,1.9));
#12024=CARTESIAN_POINT('',(-1.21,-2.4,2.));
#12025=CARTESIAN_POINT('Origin',(-1.,-2.4,2.));
#12026=CARTESIAN_POINT('',(-1.21,-2.4,2.8));
#12027=CARTESIAN_POINT('',(-1.21,-2.4,1.9));
#12028=CARTESIAN_POINT('Origin',(-1.,-2.4,2.8));
#12029=CARTESIAN_POINT('Origin',(23.,2.4,1.9));
#12030=CARTESIAN_POINT('',(22.79,2.4,2.));
#12031=CARTESIAN_POINT('Origin',(23.,2.4,2.));
#12032=CARTESIAN_POINT('',(22.79,2.4,2.8));
#12033=CARTESIAN_POINT('',(22.79,2.4,1.9));
#12034=CARTESIAN_POINT('Origin',(23.,2.4,2.8));
#12035=CARTESIAN_POINT('Origin',(19.5,-3.5,1.9));
#12036=CARTESIAN_POINT('',(19.225,-3.5,2.));
#12037=CARTESIAN_POINT('Origin',(19.5,-3.5,2.));
#12038=CARTESIAN_POINT('',(19.225,-3.5,2.8));
#12039=CARTESIAN_POINT('',(19.225,-3.5,1.9));
#12040=CARTESIAN_POINT('Origin',(19.5,-3.5,2.8));
#12041=CARTESIAN_POINT('Origin',(2.5,3.5,1.9));
#12042=CARTESIAN_POINT('',(2.225,3.5,2.));
#12043=CARTESIAN_POINT('Origin',(2.5,3.5,2.));
#12044=CARTESIAN_POINT('',(2.225,3.5,2.8));
#12045=CARTESIAN_POINT('',(2.225,3.5,1.9));
#12046=CARTESIAN_POINT('Origin',(2.5,3.5,2.8));
#12047=CARTESIAN_POINT('Origin',(2.5,-3.5,1.9));
#12048=CARTESIAN_POINT('',(2.225,-3.5,2.));
#12049=CARTESIAN_POINT('Origin',(2.5,-3.5,2.));
#12050=CARTESIAN_POINT('',(2.225,-3.5,2.8));
#12051=CARTESIAN_POINT('',(2.225,-3.5,1.9));
#12052=CARTESIAN_POINT('Origin',(2.5,-3.5,2.8));
#12053=CARTESIAN_POINT('Origin',(19.5,3.5,1.9));
#12054=CARTESIAN_POINT('',(19.225,3.5,2.));
#12055=CARTESIAN_POINT('Origin',(19.5,3.5,2.));
#12056=CARTESIAN_POINT('',(19.225,3.5,2.8));
#12057=CARTESIAN_POINT('',(19.225,3.5,1.9));
#12058=CARTESIAN_POINT('Origin',(19.5,3.5,2.8));
#12059=CARTESIAN_POINT('Origin',(14.,0.,1.9));
#12060=CARTESIAN_POINT('',(13.835,-2.02066721859312E-17,2.));
#12061=CARTESIAN_POINT('Origin',(14.,0.,2.));
#12062=CARTESIAN_POINT('',(13.835,2.02066721859312E-17,2.8));
#12063=CARTESIAN_POINT('',(13.835,-2.02066721859312E-17,1.9));
#12064=CARTESIAN_POINT('Origin',(14.,0.,2.8));
#12065=CARTESIAN_POINT('Origin',(8.,0.,1.9));
#12066=CARTESIAN_POINT('',(7.835,-2.02066721859312E-17,2.));
#12067=CARTESIAN_POINT('Origin',(8.,0.,2.));
#12068=CARTESIAN_POINT('',(7.835,2.02066721859312E-17,2.8));
#12069=CARTESIAN_POINT('',(7.835,-2.02066721859312E-17,1.9));
#12070=CARTESIAN_POINT('Origin',(8.,0.,2.8));
#12071=CARTESIAN_POINT('Origin',(2.,0.,1.9));
#12072=CARTESIAN_POINT('',(1.835,-2.02066721859313E-17,2.));
#12073=CARTESIAN_POINT('Origin',(2.,0.,2.));
#12074=CARTESIAN_POINT('',(1.835,2.02066721859313E-17,2.8));
#12075=CARTESIAN_POINT('',(1.835,-2.02066721859313E-17,1.9));
#12076=CARTESIAN_POINT('Origin',(2.,0.,2.8));
#12077=CARTESIAN_POINT('Origin',(20.,0.,1.9));
#12078=CARTESIAN_POINT('',(19.835,-2.02066721859312E-17,2.));
#12079=CARTESIAN_POINT('Origin',(20.,0.,2.));
#12080=CARTESIAN_POINT('',(19.835,2.02066721859312E-17,2.8));
#12081=CARTESIAN_POINT('',(19.835,-2.02066721859312E-17,1.9));
#12082=CARTESIAN_POINT('Origin',(20.,0.,2.8));
#12083=CARTESIAN_POINT('Origin',(24.,5.,2.));
#12084=CARTESIAN_POINT('',(24.,5.,2.));
#12085=CARTESIAN_POINT('',(-2.,5.,2.));
#12086=CARTESIAN_POINT('',(24.,5.,2.));
#12087=CARTESIAN_POINT('',(-2.,5.,2.8));
#12088=CARTESIAN_POINT('',(-2.,5.,2.));
#12089=CARTESIAN_POINT('',(24.,5.,2.8));
#12090=CARTESIAN_POINT('',(24.,5.,2.8));
#12091=CARTESIAN_POINT('',(24.,5.,2.));
#12092=CARTESIAN_POINT('Origin',(24.,-5.,2.));
#12093=CARTESIAN_POINT('',(24.,-5.,2.));
#12094=CARTESIAN_POINT('',(24.,-5.,2.));
#12095=CARTESIAN_POINT('',(24.,-5.,2.8));
#12096=CARTESIAN_POINT('',(24.,-5.,2.8));
#12097=CARTESIAN_POINT('',(24.,-5.,2.));
#12098=CARTESIAN_POINT('Origin',(-2.,-5.,2.));
#12099=CARTESIAN_POINT('',(-2.,-5.,2.));
#12100=CARTESIAN_POINT('',(-2.,-5.,2.));
#12101=CARTESIAN_POINT('',(-2.,-5.,2.8));
#12102=CARTESIAN_POINT('',(-2.,-5.,2.8));
#12103=CARTESIAN_POINT('',(-2.,-5.,2.));
#12104=CARTESIAN_POINT('Origin',(-2.,5.,2.));
#12105=CARTESIAN_POINT('',(-2.,5.,2.));
#12106=CARTESIAN_POINT('',(-2.,5.,2.8));
#12107=CARTESIAN_POINT('Origin',(11.,0.,2.8));
#12108=CARTESIAN_POINT('Origin',(11.,0.,2.));
#14417=UNCERTAINTY_MEASURE_WITH_UNIT(LENGTH_MEASURE(0.001),#14479,
'DISTANCE_ACCURACY_VALUE',
'Maximum model space distance between geometric entities at asserted c
onnectivities');
#14446=UNCERTAINTY_MEASURE_WITH_UNIT(LENGTH_MEASURE(0.001),#14479,
'DISTANCE_ACCURACY_VALUE',
'Maximum model space distance between geometric entities at asserted c
onnectivities');
#14449=(
GEOMETRIC_REPRESENTATION_CONTEXT(3)
GLOBAL_UNCERTAINTY_ASSIGNED_CONTEXT((#14417))
GLOBAL_UNIT_ASSIGNED_CONTEXT((#14479,#14481,#14482))
REPRESENTATION_CONTEXT('','3D')
);
#14478=(
GEOMETRIC_REPRESENTATION_CONTEXT(3)
GLOBAL_UNCERTAINTY_ASSIGNED_CONTEXT((#14446))
GLOBAL_UNIT_ASSIGNED_CONTEXT((#14479,#14481,#14482))
REPRESENTATION_CONTEXT('','3D')
);
#14479=(
LENGTH_UNIT()
NAMED_UNIT(*)
SI_UNIT(.CENTI.,.METRE.)
);
#14481=(
NAMED_UNIT(*)
PLANE_ANGLE_UNIT()
SI_UNIT($,.RADIAN.)
);
#14482=(
NAMED_UNIT(*)
SI_UNIT($,.STERADIAN.)
SOLID_ANGLE_UNIT()
);
#14485=SHAPE_DEFINITION_REPRESENTATION(#14516,#14605);
#14516=PRODUCT_DEFINITION_SHAPE('',$,#14637);
#14605=SHAPE_REPRESENTATION('',(#8921),#14449);
#14634=PRODUCT_DEFINITION_CONTEXT('part definition',#14729,'design');
#14637=PRODUCT_DEFINITION('Base plate','Base plate',#14668,#14634);
#14668=PRODUCT_DEFINITION_FORMATION('',$,#14733);
#14729=APPLICATION_CONTEXT(
'Core Data for Automotive Mechanical Design Process');
#14730=PRODUCT_CONTEXT('part definition',#14729,'mechanical');
#14733=PRODUCT('Base plate','Base plate','Base plate',(#14730));
#14804=COLOUR_RGB('Dark Blue',0.08,0.2,0.34);
#14805=FILL_AREA_STYLE_COLOUR('',#14804);
#14806=FILL_AREA_STYLE('',(#14805));
#14807=SURFACE_STYLE_FILL_AREA(#14806);
#14808=SURFACE_SIDE_STYLE('',(#14807));
#14809=SURFACE_STYLE_USAGE(.BOTH.,#14808);
#14810=PRESENTATION_STYLE_ASSIGNMENT((#14809));
ENDSEC;
END-ISO-10303-21;
